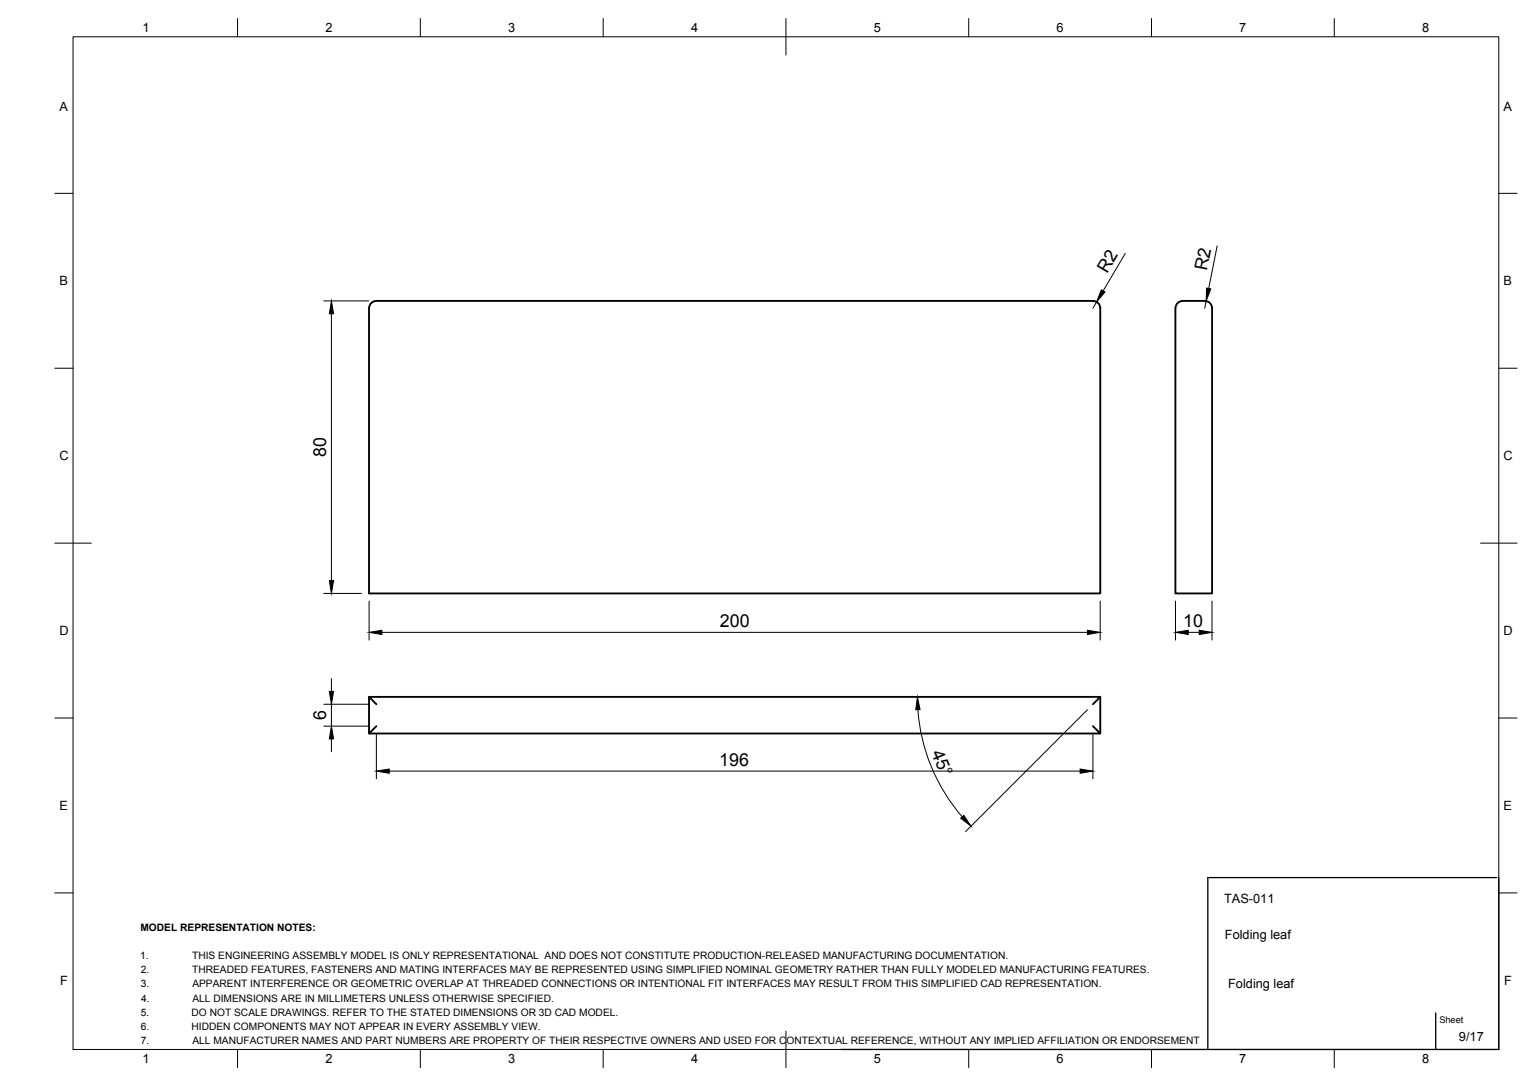
ISO-10303-21;
HEADER;
/* Generated by software containing ST-Developer
 * from STEP Tools, Inc. (www.steptools.com) 
 */

FILE_DESCRIPTION(
/* description */ (
'Independent manual bench leaf bending machine,200mm work width. Fabri
cated welded frame and folding leaf, repeated bushed and fully retaine
d hinge hardware, two handles with bonded grips, beveled clamping beam
 and modeledM12 clamp screws.2mm omitted-workpiece assembly reference 
gap, not a capacity claim. Native135deg hinge travel. Weld sizing, pro
duction fits, material condition, bending capacity, strength and life 
unassigned.'),
/* implementation_level */ '2;1');

FILE_NAME(
/* name */ 'Folding leaf.step',
/* time_stamp */ '2026-11-14T09:11:34-08:00',
/* author */ (''),
/* organization */ (''),
/* preprocessor_version */ 'ST-DEVELOPER v20.2',
/* originating_system */ 'Autodesk Translation Framework v15.17.0.0',
/* authorisation */ '');

FILE_SCHEMA (('AUTOMOTIVE_DESIGN { 1 0 10303 214 3 1 1 }'));
ENDSEC;

DATA;
#10=MECHANICAL_DESIGN_GEOMETRIC_PRESENTATION_REPRESENTATION('',(#449),#37701);
#404=ELLIPSE('',#4421,2.82842712474618,2.);
#405=ELLIPSE('',#4422,2.82842712474618,2.);
#406=ELLIPSE('',#4424,2.8284271247462,2.);
#407=ELLIPSE('',#4426,2.8284271247462,2.);
#413=SHAPE_REPRESENTATION_RELATIONSHIP('SRR','None',#37782,#431);
#431=ADVANCED_BREP_SHAPE_REPRESENTATION('',(#467),#37686);
#449=STYLED_ITEM('',(#37881),#467);
#467=MANIFOLD_SOLID_BREP('Body1',#4147);
#534=PLANE('',#4428);
#535=PLANE('',#4429);
#536=PLANE('',#4430);
#537=PLANE('',#4431);
#538=PLANE('',#4432);
#539=PLANE('',#4433);
#632=FACE_OUTER_BOUND('',#860,.T.);
#633=FACE_OUTER_BOUND('',#861,.T.);
#634=FACE_OUTER_BOUND('',#862,.T.);
#635=FACE_OUTER_BOUND('',#863,.T.);
#636=FACE_OUTER_BOUND('',#864,.T.);
#637=FACE_OUTER_BOUND('',#865,.T.);
#638=FACE_OUTER_BOUND('',#866,.T.);
#639=FACE_OUTER_BOUND('',#867,.T.);
#640=FACE_OUTER_BOUND('',#868,.T.);
#641=FACE_OUTER_BOUND('',#869,.T.);
#860=EDGE_LOOP('',(#2783,#2784,#2785,#2786));
#861=EDGE_LOOP('',(#2787,#2788,#2789,#2790));
#862=EDGE_LOOP('',(#2791,#2792,#2793,#2794));
#863=EDGE_LOOP('',(#2795,#2796,#2797,#2798));
#864=EDGE_LOOP('',(#2799,#2800,#2801,#2802));
#865=EDGE_LOOP('',(#2803,#2804,#2805,#2806));
#866=EDGE_LOOP('',(#2807,#2808,#2809,#2810));
#867=EDGE_LOOP('',(#2811,#2812,#2813,#2814));
#868=EDGE_LOOP('',(#2815,#2816,#2817,#2818));
#869=EDGE_LOOP('',(#2819,#2820,#2821,#2822));
#1108=LINE('',#5806,#1357);
#1109=LINE('',#5810,#1358);
#1110=LINE('',#5814,#1359);
#1111=LINE('',#5816,#1360);
#1112=LINE('',#5820,#1361);
#1113=LINE('',#5822,#1362);
#1114=LINE('',#5825,#1363);
#1115=LINE('',#5826,#1364);
#1116=LINE('',#5829,#1365);
#1117=LINE('',#5831,#1366);
#1118=LINE('',#5832,#1367);
#1119=LINE('',#5835,#1368);
#1120=LINE('',#5836,#1369);
#1121=LINE('',#5840,#1370);
#1122=LINE('',#5841,#1371);
#1123=LINE('',#5843,#1372);
#1357=VECTOR('',#4875,10.);
#1358=VECTOR('',#4878,10.);
#1359=VECTOR('',#4883,10.);
#1360=VECTOR('',#4884,10.);
#1361=VECTOR('',#4889,10.);
#1362=VECTOR('',#4890,10.);
#1363=VECTOR('',#4895,10.);
#1364=VECTOR('',#4896,10.);
#1365=VECTOR('',#4899,10.);
#1366=VECTOR('',#4900,10.);
#1367=VECTOR('',#4901,10.);
#1368=VECTOR('',#4904,10.);
#1369=VECTOR('',#4905,10.);
#1370=VECTOR('',#4910,10.);
#1371=VECTOR('',#4911,10.);
#1372=VECTOR('',#4914,10.);
#1685=VERTEX_POINT('',#5804);
#1686=VERTEX_POINT('',#5805);
#1687=VERTEX_POINT('',#5807);
#1688=VERTEX_POINT('',#5809);
#1689=VERTEX_POINT('',#5813);
#1690=VERTEX_POINT('',#5815);
#1691=VERTEX_POINT('',#5819);
#1692=VERTEX_POINT('',#5821);
#1693=VERTEX_POINT('',#5828);
#1694=VERTEX_POINT('',#5830);
#1695=VERTEX_POINT('',#5834);
#1696=VERTEX_POINT('',#5839);
#2125=EDGE_CURVE('',#1685,#1686,#1108,.T.);
#2126=EDGE_CURVE('',#1686,#1687,#404,.T.);
#2127=EDGE_CURVE('',#1687,#1688,#1109,.T.);
#2128=EDGE_CURVE('',#1688,#1685,#405,.T.);
#2129=EDGE_CURVE('',#1689,#1687,#1110,.T.);
#2130=EDGE_CURVE('',#1686,#1690,#1111,.T.);
#2131=EDGE_CURVE('',#1690,#1689,#406,.T.);
#2132=EDGE_CURVE('',#1691,#1685,#1112,.T.);
#2133=EDGE_CURVE('',#1688,#1692,#1113,.T.);
#2134=EDGE_CURVE('',#1692,#1691,#407,.T.);
#2135=EDGE_CURVE('',#1692,#1689,#1114,.T.);
#2136=EDGE_CURVE('',#1690,#1691,#1115,.T.);
#2137=EDGE_CURVE('',#1688,#1693,#1116,.T.);
#2138=EDGE_CURVE('',#1693,#1694,#1117,.T.);
#2139=EDGE_CURVE('',#1692,#1694,#1118,.T.);
#2140=EDGE_CURVE('',#1695,#1687,#1119,.T.);
#2141=EDGE_CURVE('',#1693,#1695,#1120,.T.);
#2142=EDGE_CURVE('',#1696,#1689,#1121,.T.);
#2143=EDGE_CURVE('',#1695,#1696,#1122,.T.);
#2144=EDGE_CURVE('',#1694,#1696,#1123,.T.);
#2783=ORIENTED_EDGE('',*,*,#2125,.T.);
#2784=ORIENTED_EDGE('',*,*,#2126,.T.);
#2785=ORIENTED_EDGE('',*,*,#2127,.T.);
#2786=ORIENTED_EDGE('',*,*,#2128,.T.);
#2787=ORIENTED_EDGE('',*,*,#2129,.T.);
#2788=ORIENTED_EDGE('',*,*,#2126,.F.);
#2789=ORIENTED_EDGE('',*,*,#2130,.T.);
#2790=ORIENTED_EDGE('',*,*,#2131,.T.);
#2791=ORIENTED_EDGE('',*,*,#2132,.T.);
#2792=ORIENTED_EDGE('',*,*,#2128,.F.);
#2793=ORIENTED_EDGE('',*,*,#2133,.T.);
#2794=ORIENTED_EDGE('',*,*,#2134,.T.);
#2795=ORIENTED_EDGE('',*,*,#2135,.T.);
#2796=ORIENTED_EDGE('',*,*,#2131,.F.);
#2797=ORIENTED_EDGE('',*,*,#2136,.T.);
#2798=ORIENTED_EDGE('',*,*,#2134,.F.);
#2799=ORIENTED_EDGE('',*,*,#2133,.F.);
#2800=ORIENTED_EDGE('',*,*,#2137,.T.);
#2801=ORIENTED_EDGE('',*,*,#2138,.T.);
#2802=ORIENTED_EDGE('',*,*,#2139,.F.);
#2803=ORIENTED_EDGE('',*,*,#2127,.F.);
#2804=ORIENTED_EDGE('',*,*,#2140,.F.);
#2805=ORIENTED_EDGE('',*,*,#2141,.F.);
#2806=ORIENTED_EDGE('',*,*,#2137,.F.);
#2807=ORIENTED_EDGE('',*,*,#2125,.F.);
#2808=ORIENTED_EDGE('',*,*,#2132,.F.);
#2809=ORIENTED_EDGE('',*,*,#2136,.F.);
#2810=ORIENTED_EDGE('',*,*,#2130,.F.);
#2811=ORIENTED_EDGE('',*,*,#2129,.F.);
#2812=ORIENTED_EDGE('',*,*,#2142,.F.);
#2813=ORIENTED_EDGE('',*,*,#2143,.F.);
#2814=ORIENTED_EDGE('',*,*,#2140,.T.);
#2815=ORIENTED_EDGE('',*,*,#2141,.T.);
#2816=ORIENTED_EDGE('',*,*,#2143,.T.);
#2817=ORIENTED_EDGE('',*,*,#2144,.F.);
#2818=ORIENTED_EDGE('',*,*,#2138,.F.);
#2819=ORIENTED_EDGE('',*,*,#2135,.F.);
#2820=ORIENTED_EDGE('',*,*,#2139,.T.);
#2821=ORIENTED_EDGE('',*,*,#2144,.T.);
#2822=ORIENTED_EDGE('',*,*,#2142,.T.);
#3823=CYLINDRICAL_SURFACE('',#4420,2.);
#3824=CYLINDRICAL_SURFACE('',#4423,2.);
#3825=CYLINDRICAL_SURFACE('',#4425,2.);
#3826=CYLINDRICAL_SURFACE('',#4427,2.);
#3962=ADVANCED_FACE('',(#632),#3823,.T.);
#3963=ADVANCED_FACE('',(#633),#3824,.T.);
#3964=ADVANCED_FACE('',(#634),#3825,.T.);
#3965=ADVANCED_FACE('',(#635),#3826,.T.);
#3966=ADVANCED_FACE('',(#636),#534,.T.);
#3967=ADVANCED_FACE('',(#637),#535,.F.);
#3968=ADVANCED_FACE('',(#638),#536,.T.);
#3969=ADVANCED_FACE('',(#639),#537,.T.);
#3970=ADVANCED_FACE('',(#640),#538,.T.);
#3971=ADVANCED_FACE('',(#641),#539,.T.);
#4147=CLOSED_SHELL('',(#3962,#3963,#3964,#3965,#3966,#3967,#3968,#3969,
#3970,#3971));
#4419=AXIS2_PLACEMENT_3D('',#5802,#4871,#4872);
#4420=AXIS2_PLACEMENT_3D('',#5803,#4873,#4874);
#4421=AXIS2_PLACEMENT_3D('',#5808,#4876,#4877);
#4422=AXIS2_PLACEMENT_3D('',#5811,#4879,#4880);
#4423=AXIS2_PLACEMENT_3D('',#5812,#4881,#4882);
#4424=AXIS2_PLACEMENT_3D('',#5817,#4885,#4886);
#4425=AXIS2_PLACEMENT_3D('',#5818,#4887,#4888);
#4426=AXIS2_PLACEMENT_3D('',#5823,#4891,#4892);
#4427=AXIS2_PLACEMENT_3D('',#5824,#4893,#4894);
#4428=AXIS2_PLACEMENT_3D('',#5827,#4897,#4898);
#4429=AXIS2_PLACEMENT_3D('',#5833,#4902,#4903);
#4430=AXIS2_PLACEMENT_3D('',#5837,#4906,#4907);
#4431=AXIS2_PLACEMENT_3D('',#5838,#4908,#4909);
#4432=AXIS2_PLACEMENT_3D('',#5842,#4912,#4913);
#4433=AXIS2_PLACEMENT_3D('',#5844,#4915,#4916);
#4871=DIRECTION('axis',(0.,0.,1.));
#4872=DIRECTION('refdir',(1.,0.,0.));
#4873=DIRECTION('center_axis',(0.,1.,0.));
#4874=DIRECTION('ref_axis',(0.707106781186546,0.,-0.707106781186549));
#4875=DIRECTION('',(0.,-1.,0.));
#4876=DIRECTION('center_axis',(0.,0.707106781186549,-0.707106781186546));
#4877=DIRECTION('ref_axis',(0.,-0.707106781186546,-0.707106781186549));
#4878=DIRECTION('',(0.,1.,0.));
#4879=DIRECTION('center_axis',(0.,-0.707106781186549,-0.707106781186546));
#4880=DIRECTION('ref_axis',(0.,-0.707106781186546,0.707106781186549));
#4881=DIRECTION('center_axis',(0.,0.,1.));
#4882=DIRECTION('ref_axis',(0.707106781186551,-0.707106781186544,0.));
#4883=DIRECTION('',(0.,0.,-1.));
#4884=DIRECTION('',(0.,0.,1.));
#4885=DIRECTION('center_axis',(0.,-0.707106781186549,-0.707106781186546));
#4886=DIRECTION('ref_axis',(0.,0.707106781186546,-0.707106781186549));
#4887=DIRECTION('center_axis',(0.,0.,1.));
#4888=DIRECTION('ref_axis',(0.707106781186548,0.707106781186548,0.));
#4889=DIRECTION('',(0.,0.,-1.));
#4890=DIRECTION('',(0.,0.,1.));
#4891=DIRECTION('center_axis',(0.,0.707106781186549,-0.707106781186546));
#4892=DIRECTION('ref_axis',(0.,-0.707106781186546,-0.707106781186549));
#4893=DIRECTION('center_axis',(0.,1.,0.));
#4894=DIRECTION('ref_axis',(0.707106781186549,0.,0.707106781186546));
#4895=DIRECTION('',(0.,-1.,0.));
#4896=DIRECTION('',(0.,1.,0.));
#4897=DIRECTION('center_axis',(0.,1.,0.));
#4898=DIRECTION('ref_axis',(-1.,0.,0.));
#4899=DIRECTION('',(-1.,0.,0.));
#4900=DIRECTION('',(0.,0.,1.));
#4901=DIRECTION('',(-1.,0.,0.));
#4902=DIRECTION('center_axis',(0.,0.,1.));
#4903=DIRECTION('ref_axis',(1.,0.,0.));
#4904=DIRECTION('',(1.,0.,0.));
#4905=DIRECTION('',(0.,-1.,0.));
#4906=DIRECTION('center_axis',(1.,0.,0.));
#4907=DIRECTION('ref_axis',(0.,1.,0.));
#4908=DIRECTION('center_axis',(0.,-1.,0.));
#4909=DIRECTION('ref_axis',(1.,0.,0.));
#4910=DIRECTION('',(1.,0.,0.));
#4911=DIRECTION('',(0.,0.,1.));
#4912=DIRECTION('center_axis',(-1.,0.,0.));
#4913=DIRECTION('ref_axis',(0.,-1.,0.));
#4914=DIRECTION('',(0.,-1.,0.));
#4915=DIRECTION('center_axis',(0.,0.,1.));
#4916=DIRECTION('ref_axis',(1.,0.,0.));
#5802=CARTESIAN_POINT('',(0.,0.,0.));
#5803=CARTESIAN_POINT('Origin',(78.,-50.,32.));
#5804=CARTESIAN_POINT('',(80.,98.,32.));
#5805=CARTESIAN_POINT('',(80.,-98.,32.));
#5806=CARTESIAN_POINT('',(80.,-50.,32.));
#5807=CARTESIAN_POINT('',(78.,-100.,30.));
#5808=CARTESIAN_POINT('Origin',(78.,-98.,32.));
#5809=CARTESIAN_POINT('',(78.,100.,30.));
#5810=CARTESIAN_POINT('',(78.,-50.,30.));
#5811=CARTESIAN_POINT('Origin',(78.,98.,32.));
#5812=CARTESIAN_POINT('Origin',(78.,-98.,30.));
#5813=CARTESIAN_POINT('',(78.,-100.,40.));
#5814=CARTESIAN_POINT('',(78.,-100.,30.));
#5815=CARTESIAN_POINT('',(80.,-98.,38.));
#5816=CARTESIAN_POINT('',(80.,-98.,30.));
#5817=CARTESIAN_POINT('Origin',(78.,-98.,38.));
#5818=CARTESIAN_POINT('Origin',(78.,98.,30.));
#5819=CARTESIAN_POINT('',(80.,98.,38.));
#5820=CARTESIAN_POINT('',(80.,98.,30.));
#5821=CARTESIAN_POINT('',(78.,100.,40.));
#5822=CARTESIAN_POINT('',(78.,100.,30.));
#5823=CARTESIAN_POINT('Origin',(78.,98.,38.));
#5824=CARTESIAN_POINT('Origin',(78.,-50.,38.));
#5825=CARTESIAN_POINT('',(78.,-50.,40.));
#5826=CARTESIAN_POINT('',(80.,-50.,38.));
#5827=CARTESIAN_POINT('Origin',(80.,100.,30.));
#5828=CARTESIAN_POINT('',(0.,100.,30.));
#5829=CARTESIAN_POINT('',(80.,100.,30.));
#5830=CARTESIAN_POINT('',(0.,100.,40.));
#5831=CARTESIAN_POINT('',(0.,100.,30.));
#5832=CARTESIAN_POINT('',(80.,100.,40.));
#5833=CARTESIAN_POINT('Origin',(40.,0.,30.));
#5834=CARTESIAN_POINT('',(0.,-100.,30.));
#5835=CARTESIAN_POINT('',(0.,-100.,30.));
#5836=CARTESIAN_POINT('',(0.,100.,30.));
#5837=CARTESIAN_POINT('Origin',(80.,-100.,30.));
#5838=CARTESIAN_POINT('Origin',(0.,-100.,30.));
#5839=CARTESIAN_POINT('',(0.,-100.,40.));
#5840=CARTESIAN_POINT('',(0.,-100.,40.));
#5841=CARTESIAN_POINT('',(0.,-100.,30.));
#5842=CARTESIAN_POINT('Origin',(0.,100.,30.));
#5843=CARTESIAN_POINT('',(0.,100.,40.));
#5844=CARTESIAN_POINT('Origin',(40.,0.,40.));
#37666=UNCERTAINTY_MEASURE_WITH_UNIT(LENGTH_MEASURE(0.01),#37702,
'DISTANCE_ACCURACY_VALUE',
'Maximum model space distance between geometric entities at asserted c
onnectivities');
#37681=UNCERTAINTY_MEASURE_WITH_UNIT(LENGTH_MEASURE(0.01),#37702,
'DISTANCE_ACCURACY_VALUE',
'Maximum model space distance between geometric entities at asserted c
onnectivities');
#37686=(
GEOMETRIC_REPRESENTATION_CONTEXT(3)
GLOBAL_UNCERTAINTY_ASSIGNED_CONTEXT((#37666))
GLOBAL_UNIT_ASSIGNED_CONTEXT((#37702,#37704,#37705))
REPRESENTATION_CONTEXT('','3D')
);
#37701=(
GEOMETRIC_REPRESENTATION_CONTEXT(3)
GLOBAL_UNCERTAINTY_ASSIGNED_CONTEXT((#37681))
GLOBAL_UNIT_ASSIGNED_CONTEXT((#37702,#37704,#37705))
REPRESENTATION_CONTEXT('','3D')
);
#37702=(
LENGTH_UNIT()
NAMED_UNIT(*)
SI_UNIT(.MILLI.,.METRE.)
);
#37704=(
NAMED_UNIT(*)
PLANE_ANGLE_UNIT()
SI_UNIT($,.RADIAN.)
);
#37705=(
NAMED_UNIT(*)
SI_UNIT($,.STERADIAN.)
SOLID_ANGLE_UNIT()
);
#37710=SHAPE_DEFINITION_REPRESENTATION(#37729,#37782);
#37729=PRODUCT_DEFINITION_SHAPE('',$,#37802);
#37782=SHAPE_REPRESENTATION('',(#4419),#37686);
#37797=PRODUCT_DEFINITION_CONTEXT('part definition',#37856,'design');
#37802=PRODUCT_DEFINITION('Folding leaf','Folding leaf',#37821,#37797);
#37821=PRODUCT_DEFINITION_FORMATION('',$,#37862);
#37856=APPLICATION_CONTEXT(
'Core Data for Automotive Mechanical Design Process');
#37857=PRODUCT_CONTEXT('part definition',#37856,'mechanical');
#37862=PRODUCT('Folding leaf','Folding leaf',$,(#37857));
#37881=PRESENTATION_STYLE_ASSIGNMENT((#37889));
#37889=SURFACE_STYLE_USAGE(.BOTH.,#37897);
#37897=SURFACE_SIDE_STYLE('',(#37905));
#37905=SURFACE_STYLE_FILL_AREA(#37913);
#37913=FILL_AREA_STYLE('Opaque(81,175,227)',(#37921));
#37921=FILL_AREA_STYLE_COLOUR('Opaque(81,175,227)',#37929);
#37929=COLOUR_RGB('Opaque(81,175,227)',0.317647058823529,0.686274509803922,
0.890196078431372);
ENDSEC;
END-ISO-10303-21;
